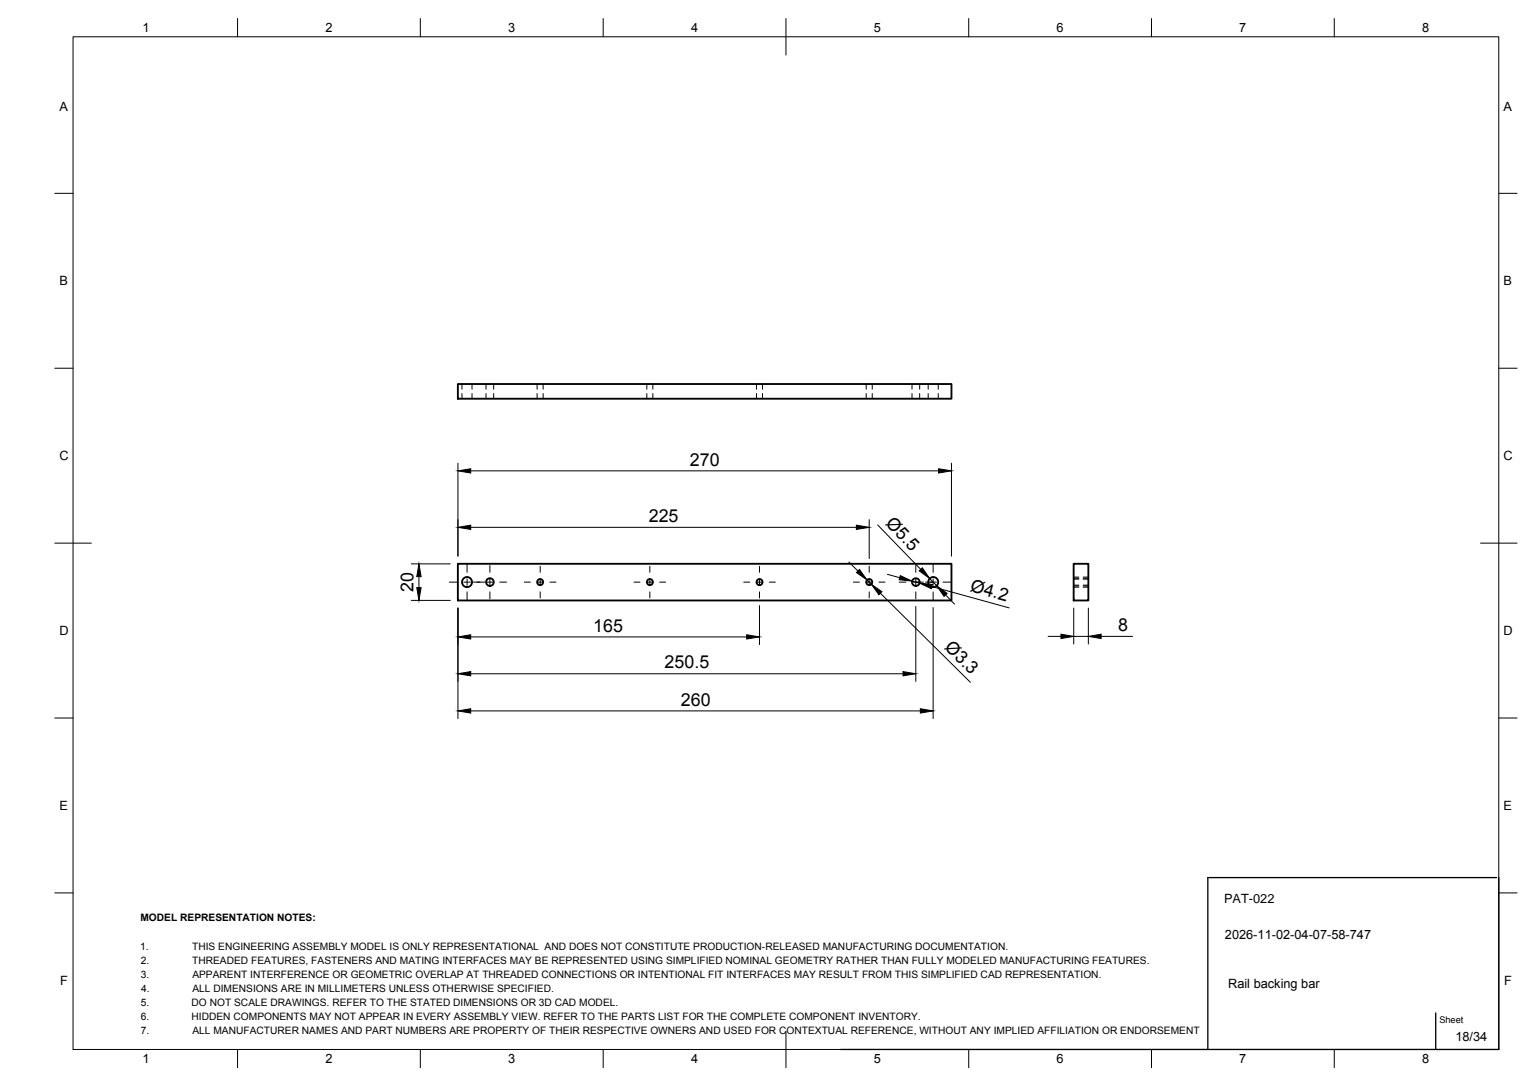
ISO-10303-21;
HEADER;
/* Generated by software containing ST-Developer
 * from STEP Tools, Inc. (www.steptools.com) 
 */

FILE_DESCRIPTION(
/* description */ ('Chute with adjustable gate'),
/* implementation_level */ '2;1');

FILE_NAME(
/* name */ 'Rail backing bar.step',
/* time_stamp */ '2026-10-27T10:52:28-07:00',
/* author */ (''),
/* organization */ (''),
/* preprocessor_version */ 'ST-DEVELOPER v20.2',
/* originating_system */ 'Autodesk Translation Framework v15.17.0.0',
/* authorisation */ '');

FILE_SCHEMA (('AUTOMOTIVE_DESIGN { 1 0 10303 214 3 1 1 }'));
ENDSEC;

DATA;
#10=MECHANICAL_DESIGN_GEOMETRIC_PRESENTATION_REPRESENTATION('',(#427),#13094);
#363=SHAPE_REPRESENTATION_RELATIONSHIP('SRR','None',#13264,#395);
#395=ADVANCED_BREP_SHAPE_REPRESENTATION('',(#459),#13073);
#427=STYLED_ITEM('',(#13481),#459);
#459=MANIFOLD_SOLID_BREP('Body1',#7610);
#520=FACE_BOUND('',#1507,.T.);
#521=FACE_BOUND('',#1508,.T.);
#522=FACE_BOUND('',#1509,.T.);
#523=FACE_BOUND('',#1510,.T.);
#524=FACE_BOUND('',#1511,.T.);
#525=FACE_BOUND('',#1512,.T.);
#526=FACE_BOUND('',#1513,.T.);
#527=FACE_BOUND('',#1514,.T.);
#528=FACE_BOUND('',#1517,.T.);
#529=FACE_BOUND('',#1518,.T.);
#530=FACE_BOUND('',#1519,.T.);
#531=FACE_BOUND('',#1520,.T.);
#532=FACE_BOUND('',#1521,.T.);
#533=FACE_BOUND('',#1522,.T.);
#534=FACE_BOUND('',#1523,.T.);
#535=FACE_BOUND('',#1524,.T.);
#688=PLANE('',#8196);
#689=PLANE('',#8197);
#690=PLANE('',#8198);
#691=PLANE('',#8199);
#692=PLANE('',#8200);
#693=PLANE('',#8201);
#1036=FACE_OUTER_BOUND('',#1497,.T.);
#1037=FACE_OUTER_BOUND('',#1498,.T.);
#1038=FACE_OUTER_BOUND('',#1499,.T.);
#1039=FACE_OUTER_BOUND('',#1500,.T.);
#1040=FACE_OUTER_BOUND('',#1501,.T.);
#1041=FACE_OUTER_BOUND('',#1502,.T.);
#1042=FACE_OUTER_BOUND('',#1503,.T.);
#1043=FACE_OUTER_BOUND('',#1504,.T.);
#1044=FACE_OUTER_BOUND('',#1505,.T.);
#1045=FACE_OUTER_BOUND('',#1506,.T.);
#1046=FACE_OUTER_BOUND('',#1515,.T.);
#1047=FACE_OUTER_BOUND('',#1516,.T.);
#1048=FACE_OUTER_BOUND('',#1525,.T.);
#1049=FACE_OUTER_BOUND('',#1526,.T.);
#1497=EDGE_LOOP('',(#5714,#5715,#5716,#5717));
#1498=EDGE_LOOP('',(#5718,#5719,#5720,#5721));
#1499=EDGE_LOOP('',(#5722,#5723,#5724,#5725));
#1500=EDGE_LOOP('',(#5726,#5727,#5728,#5729));
#1501=EDGE_LOOP('',(#5730,#5731,#5732,#5733));
#1502=EDGE_LOOP('',(#5734,#5735,#5736,#5737));
#1503=EDGE_LOOP('',(#5738,#5739,#5740,#5741));
#1504=EDGE_LOOP('',(#5742,#5743,#5744,#5745));
#1505=EDGE_LOOP('',(#5746,#5747,#5748,#5749));
#1506=EDGE_LOOP('',(#5750,#5751,#5752,#5753));
#1507=EDGE_LOOP('',(#5754));
#1508=EDGE_LOOP('',(#5755));
#1509=EDGE_LOOP('',(#5756));
#1510=EDGE_LOOP('',(#5757));
#1511=EDGE_LOOP('',(#5758));
#1512=EDGE_LOOP('',(#5759));
#1513=EDGE_LOOP('',(#5760));
#1514=EDGE_LOOP('',(#5761));
#1515=EDGE_LOOP('',(#5762,#5763,#5764,#5765));
#1516=EDGE_LOOP('',(#5766,#5767,#5768,#5769));
#1517=EDGE_LOOP('',(#5770));
#1518=EDGE_LOOP('',(#5771));
#1519=EDGE_LOOP('',(#5772));
#1520=EDGE_LOOP('',(#5773));
#1521=EDGE_LOOP('',(#5774));
#1522=EDGE_LOOP('',(#5775));
#1523=EDGE_LOOP('',(#5776));
#1524=EDGE_LOOP('',(#5777));
#1525=EDGE_LOOP('',(#5778,#5779,#5780,#5781));
#1526=EDGE_LOOP('',(#5782,#5783,#5784,#5785));
#2076=LINE('',#11481,#2853);
#2077=LINE('',#11487,#2854);
#2078=LINE('',#11493,#2855);
#2079=LINE('',#11499,#2856);
#2080=LINE('',#11505,#2857);
#2081=LINE('',#11511,#2858);
#2082=LINE('',#11517,#2859);
#2083=LINE('',#11523,#2860);
#2084=LINE('',#11528,#2861);
#2085=LINE('',#11530,#2862);
#2086=LINE('',#11532,#2863);
#2087=LINE('',#11533,#2864);
#2088=LINE('',#11536,#2865);
#2089=LINE('',#11538,#2866);
#2090=LINE('',#11539,#2867);
#2091=LINE('',#11542,#2868);
#2092=LINE('',#11544,#2869);
#2093=LINE('',#11545,#2870);
#2094=LINE('',#11547,#2871);
#2095=LINE('',#11548,#2872);
#2853=VECTOR('',#9290,0.210000000000001);
#2854=VECTOR('',#9297,0.21);
#2855=VECTOR('',#9304,0.164999999999999);
#2856=VECTOR('',#9311,0.164999999999999);
#2857=VECTOR('',#9318,0.164999999999999);
#2858=VECTOR('',#9325,0.164999999999999);
#2859=VECTOR('',#9332,0.275);
#2860=VECTOR('',#9339,0.274999999999999);
#2861=VECTOR('',#9344,1.);
#2862=VECTOR('',#9345,1.);
#2863=VECTOR('',#9346,1.);
#2864=VECTOR('',#9347,1.);
#2865=VECTOR('',#9350,1.);
#2866=VECTOR('',#9351,1.);
#2867=VECTOR('',#9352,1.);
#2868=VECTOR('',#9355,1.);
#2869=VECTOR('',#9356,1.);
#2870=VECTOR('',#9357,1.);
#2871=VECTOR('',#9360,1.);
#2872=VECTOR('',#9361,1.);
#3462=CIRCLE('',#8173,0.210000000000001);
#3463=CIRCLE('',#8174,0.210000000000001);
#3464=CIRCLE('',#8176,0.21);
#3465=CIRCLE('',#8177,0.21);
#3466=CIRCLE('',#8179,0.164999999999999);
#3467=CIRCLE('',#8180,0.164999999999999);
#3468=CIRCLE('',#8182,0.164999999999999);
#3469=CIRCLE('',#8183,0.164999999999999);
#3470=CIRCLE('',#8185,0.164999999999999);
#3471=CIRCLE('',#8186,0.164999999999999);
#3472=CIRCLE('',#8188,0.164999999999999);
#3473=CIRCLE('',#8189,0.164999999999999);
#3474=CIRCLE('',#8191,0.275);
#3475=CIRCLE('',#8192,0.275);
#3476=CIRCLE('',#8194,0.274999999999999);
#3477=CIRCLE('',#8195,0.274999999999999);
#3769=VERTEX_POINT('',#11478);
#3770=VERTEX_POINT('',#11480);
#3771=VERTEX_POINT('',#11484);
#3772=VERTEX_POINT('',#11486);
#3773=VERTEX_POINT('',#11490);
#3774=VERTEX_POINT('',#11492);
#3775=VERTEX_POINT('',#11496);
#3776=VERTEX_POINT('',#11498);
#3777=VERTEX_POINT('',#11502);
#3778=VERTEX_POINT('',#11504);
#3779=VERTEX_POINT('',#11508);
#3780=VERTEX_POINT('',#11510);
#3781=VERTEX_POINT('',#11514);
#3782=VERTEX_POINT('',#11516);
#3783=VERTEX_POINT('',#11520);
#3784=VERTEX_POINT('',#11522);
#3785=VERTEX_POINT('',#11526);
#3786=VERTEX_POINT('',#11527);
#3787=VERTEX_POINT('',#11529);
#3788=VERTEX_POINT('',#11531);
#3789=VERTEX_POINT('',#11535);
#3790=VERTEX_POINT('',#11537);
#3791=VERTEX_POINT('',#11541);
#3792=VERTEX_POINT('',#11543);
#4490=EDGE_CURVE('',#3769,#3769,#3462,.T.);
#4491=EDGE_CURVE('',#3769,#3770,#2076,.T.);
#4492=EDGE_CURVE('',#3770,#3770,#3463,.T.);
#4493=EDGE_CURVE('',#3771,#3771,#3464,.T.);
#4494=EDGE_CURVE('',#3771,#3772,#2077,.T.);
#4495=EDGE_CURVE('',#3772,#3772,#3465,.T.);
#4496=EDGE_CURVE('',#3773,#3773,#3466,.T.);
#4497=EDGE_CURVE('',#3773,#3774,#2078,.T.);
#4498=EDGE_CURVE('',#3774,#3774,#3467,.T.);
#4499=EDGE_CURVE('',#3775,#3775,#3468,.T.);
#4500=EDGE_CURVE('',#3775,#3776,#2079,.T.);
#4501=EDGE_CURVE('',#3776,#3776,#3469,.T.);
#4502=EDGE_CURVE('',#3777,#3777,#3470,.T.);
#4503=EDGE_CURVE('',#3777,#3778,#2080,.T.);
#4504=EDGE_CURVE('',#3778,#3778,#3471,.T.);
#4505=EDGE_CURVE('',#3779,#3779,#3472,.T.);
#4506=EDGE_CURVE('',#3779,#3780,#2081,.T.);
#4507=EDGE_CURVE('',#3780,#3780,#3473,.T.);
#4508=EDGE_CURVE('',#3781,#3781,#3474,.T.);
#4509=EDGE_CURVE('',#3781,#3782,#2082,.T.);
#4510=EDGE_CURVE('',#3782,#3782,#3475,.T.);
#4511=EDGE_CURVE('',#3783,#3783,#3476,.T.);
#4512=EDGE_CURVE('',#3783,#3784,#2083,.T.);
#4513=EDGE_CURVE('',#3784,#3784,#3477,.T.);
#4514=EDGE_CURVE('',#3785,#3786,#2084,.T.);
#4515=EDGE_CURVE('',#3786,#3787,#2085,.T.);
#4516=EDGE_CURVE('',#3788,#3787,#2086,.T.);
#4517=EDGE_CURVE('',#3785,#3788,#2087,.T.);
#4518=EDGE_CURVE('',#3789,#3785,#2088,.T.);
#4519=EDGE_CURVE('',#3790,#3788,#2089,.T.);
#4520=EDGE_CURVE('',#3789,#3790,#2090,.T.);
#4521=EDGE_CURVE('',#3791,#3789,#2091,.T.);
#4522=EDGE_CURVE('',#3792,#3790,#2092,.T.);
#4523=EDGE_CURVE('',#3791,#3792,#2093,.T.);
#4524=EDGE_CURVE('',#3786,#3791,#2094,.T.);
#4525=EDGE_CURVE('',#3787,#3792,#2095,.T.);
#5714=ORIENTED_EDGE('',*,*,#4490,.F.);
#5715=ORIENTED_EDGE('',*,*,#4491,.T.);
#5716=ORIENTED_EDGE('',*,*,#4492,.F.);
#5717=ORIENTED_EDGE('',*,*,#4491,.F.);
#5718=ORIENTED_EDGE('',*,*,#4493,.F.);
#5719=ORIENTED_EDGE('',*,*,#4494,.T.);
#5720=ORIENTED_EDGE('',*,*,#4495,.F.);
#5721=ORIENTED_EDGE('',*,*,#4494,.F.);
#5722=ORIENTED_EDGE('',*,*,#4496,.F.);
#5723=ORIENTED_EDGE('',*,*,#4497,.T.);
#5724=ORIENTED_EDGE('',*,*,#4498,.F.);
#5725=ORIENTED_EDGE('',*,*,#4497,.F.);
#5726=ORIENTED_EDGE('',*,*,#4499,.F.);
#5727=ORIENTED_EDGE('',*,*,#4500,.T.);
#5728=ORIENTED_EDGE('',*,*,#4501,.F.);
#5729=ORIENTED_EDGE('',*,*,#4500,.F.);
#5730=ORIENTED_EDGE('',*,*,#4502,.F.);
#5731=ORIENTED_EDGE('',*,*,#4503,.T.);
#5732=ORIENTED_EDGE('',*,*,#4504,.F.);
#5733=ORIENTED_EDGE('',*,*,#4503,.F.);
#5734=ORIENTED_EDGE('',*,*,#4505,.F.);
#5735=ORIENTED_EDGE('',*,*,#4506,.T.);
#5736=ORIENTED_EDGE('',*,*,#4507,.F.);
#5737=ORIENTED_EDGE('',*,*,#4506,.F.);
#5738=ORIENTED_EDGE('',*,*,#4508,.F.);
#5739=ORIENTED_EDGE('',*,*,#4509,.T.);
#5740=ORIENTED_EDGE('',*,*,#4510,.F.);
#5741=ORIENTED_EDGE('',*,*,#4509,.F.);
#5742=ORIENTED_EDGE('',*,*,#4511,.F.);
#5743=ORIENTED_EDGE('',*,*,#4512,.T.);
#5744=ORIENTED_EDGE('',*,*,#4513,.F.);
#5745=ORIENTED_EDGE('',*,*,#4512,.F.);
#5746=ORIENTED_EDGE('',*,*,#4514,.T.);
#5747=ORIENTED_EDGE('',*,*,#4515,.T.);
#5748=ORIENTED_EDGE('',*,*,#4516,.F.);
#5749=ORIENTED_EDGE('',*,*,#4517,.F.);
#5750=ORIENTED_EDGE('',*,*,#4518,.T.);
#5751=ORIENTED_EDGE('',*,*,#4517,.T.);
#5752=ORIENTED_EDGE('',*,*,#4519,.F.);
#5753=ORIENTED_EDGE('',*,*,#4520,.F.);
#5754=ORIENTED_EDGE('',*,*,#4498,.T.);
#5755=ORIENTED_EDGE('',*,*,#4501,.T.);
#5756=ORIENTED_EDGE('',*,*,#4504,.T.);
#5757=ORIENTED_EDGE('',*,*,#4507,.T.);
#5758=ORIENTED_EDGE('',*,*,#4510,.T.);
#5759=ORIENTED_EDGE('',*,*,#4513,.T.);
#5760=ORIENTED_EDGE('',*,*,#4495,.T.);
#5761=ORIENTED_EDGE('',*,*,#4492,.T.);
#5762=ORIENTED_EDGE('',*,*,#4521,.T.);
#5763=ORIENTED_EDGE('',*,*,#4520,.T.);
#5764=ORIENTED_EDGE('',*,*,#4522,.F.);
#5765=ORIENTED_EDGE('',*,*,#4523,.F.);
#5766=ORIENTED_EDGE('',*,*,#4524,.T.);
#5767=ORIENTED_EDGE('',*,*,#4523,.T.);
#5768=ORIENTED_EDGE('',*,*,#4525,.F.);
#5769=ORIENTED_EDGE('',*,*,#4515,.F.);
#5770=ORIENTED_EDGE('',*,*,#4496,.T.);
#5771=ORIENTED_EDGE('',*,*,#4499,.T.);
#5772=ORIENTED_EDGE('',*,*,#4502,.T.);
#5773=ORIENTED_EDGE('',*,*,#4505,.T.);
#5774=ORIENTED_EDGE('',*,*,#4508,.T.);
#5775=ORIENTED_EDGE('',*,*,#4511,.T.);
#5776=ORIENTED_EDGE('',*,*,#4493,.T.);
#5777=ORIENTED_EDGE('',*,*,#4490,.T.);
#5778=ORIENTED_EDGE('',*,*,#4525,.T.);
#5779=ORIENTED_EDGE('',*,*,#4522,.T.);
#5780=ORIENTED_EDGE('',*,*,#4519,.T.);
#5781=ORIENTED_EDGE('',*,*,#4516,.T.);
#5782=ORIENTED_EDGE('',*,*,#4524,.F.);
#5783=ORIENTED_EDGE('',*,*,#4514,.F.);
#5784=ORIENTED_EDGE('',*,*,#4518,.F.);
#5785=ORIENTED_EDGE('',*,*,#4521,.F.);
#7130=CYLINDRICAL_SURFACE('',#8172,0.210000000000001);
#7131=CYLINDRICAL_SURFACE('',#8175,0.21);
#7132=CYLINDRICAL_SURFACE('',#8178,0.164999999999999);
#7133=CYLINDRICAL_SURFACE('',#8181,0.164999999999999);
#7134=CYLINDRICAL_SURFACE('',#8184,0.164999999999999);
#7135=CYLINDRICAL_SURFACE('',#8187,0.164999999999999);
#7136=CYLINDRICAL_SURFACE('',#8190,0.275);
#7137=CYLINDRICAL_SURFACE('',#8193,0.274999999999999);
#7304=ADVANCED_FACE('',(#1036),#7130,.F.);
#7305=ADVANCED_FACE('',(#1037),#7131,.F.);
#7306=ADVANCED_FACE('',(#1038),#7132,.F.);
#7307=ADVANCED_FACE('',(#1039),#7133,.F.);
#7308=ADVANCED_FACE('',(#1040),#7134,.F.);
#7309=ADVANCED_FACE('',(#1041),#7135,.F.);
#7310=ADVANCED_FACE('',(#1042),#7136,.F.);
#7311=ADVANCED_FACE('',(#1043),#7137,.F.);
#7312=ADVANCED_FACE('',(#1044),#688,.T.);
#7313=ADVANCED_FACE('',(#1045,#520,#521,#522,#523,#524,#525,#526,#527),
#689,.T.);
#7314=ADVANCED_FACE('',(#1046),#690,.T.);
#7315=ADVANCED_FACE('',(#1047,#528,#529,#530,#531,#532,#533,#534,#535),
#691,.T.);
#7316=ADVANCED_FACE('',(#1048),#692,.T.);
#7317=ADVANCED_FACE('',(#1049),#693,.F.);
#7610=CLOSED_SHELL('',(#7304,#7305,#7306,#7307,#7308,#7309,#7310,#7311,
#7312,#7313,#7314,#7315,#7316,#7317));
#8171=AXIS2_PLACEMENT_3D('',#11476,#9284,#9285);
#8172=AXIS2_PLACEMENT_3D('',#11477,#9286,#9287);
#8173=AXIS2_PLACEMENT_3D('',#11479,#9288,#9289);
#8174=AXIS2_PLACEMENT_3D('',#11482,#9291,#9292);
#8175=AXIS2_PLACEMENT_3D('',#11483,#9293,#9294);
#8176=AXIS2_PLACEMENT_3D('',#11485,#9295,#9296);
#8177=AXIS2_PLACEMENT_3D('',#11488,#9298,#9299);
#8178=AXIS2_PLACEMENT_3D('',#11489,#9300,#9301);
#8179=AXIS2_PLACEMENT_3D('',#11491,#9302,#9303);
#8180=AXIS2_PLACEMENT_3D('',#11494,#9305,#9306);
#8181=AXIS2_PLACEMENT_3D('',#11495,#9307,#9308);
#8182=AXIS2_PLACEMENT_3D('',#11497,#9309,#9310);
#8183=AXIS2_PLACEMENT_3D('',#11500,#9312,#9313);
#8184=AXIS2_PLACEMENT_3D('',#11501,#9314,#9315);
#8185=AXIS2_PLACEMENT_3D('',#11503,#9316,#9317);
#8186=AXIS2_PLACEMENT_3D('',#11506,#9319,#9320);
#8187=AXIS2_PLACEMENT_3D('',#11507,#9321,#9322);
#8188=AXIS2_PLACEMENT_3D('',#11509,#9323,#9324);
#8189=AXIS2_PLACEMENT_3D('',#11512,#9326,#9327);
#8190=AXIS2_PLACEMENT_3D('',#11513,#9328,#9329);
#8191=AXIS2_PLACEMENT_3D('',#11515,#9330,#9331);
#8192=AXIS2_PLACEMENT_3D('',#11518,#9333,#9334);
#8193=AXIS2_PLACEMENT_3D('',#11519,#9335,#9336);
#8194=AXIS2_PLACEMENT_3D('',#11521,#9337,#9338);
#8195=AXIS2_PLACEMENT_3D('',#11524,#9340,#9341);
#8196=AXIS2_PLACEMENT_3D('',#11525,#9342,#9343);
#8197=AXIS2_PLACEMENT_3D('',#11534,#9348,#9349);
#8198=AXIS2_PLACEMENT_3D('',#11540,#9353,#9354);
#8199=AXIS2_PLACEMENT_3D('',#11546,#9358,#9359);
#8200=AXIS2_PLACEMENT_3D('',#11549,#9362,#9363);
#8201=AXIS2_PLACEMENT_3D('',#11550,#9364,#9365);
#9284=DIRECTION('axis',(0.,0.,1.));
#9285=DIRECTION('refdir',(1.,0.,0.));
#9286=DIRECTION('center_axis',(1.,0.,0.));
#9287=DIRECTION('ref_axis',(0.,0.,-1.));
#9288=DIRECTION('center_axis',(1.,0.,0.));
#9289=DIRECTION('ref_axis',(0.,0.,-1.));
#9290=DIRECTION('',(1.,0.,0.));
#9291=DIRECTION('center_axis',(-1.,0.,0.));
#9292=DIRECTION('ref_axis',(0.,0.,-1.));
#9293=DIRECTION('center_axis',(1.,0.,0.));
#9294=DIRECTION('ref_axis',(0.,0.,-1.));
#9295=DIRECTION('center_axis',(1.,0.,0.));
#9296=DIRECTION('ref_axis',(0.,0.,-1.));
#9297=DIRECTION('',(1.,0.,0.));
#9298=DIRECTION('center_axis',(-1.,0.,0.));
#9299=DIRECTION('ref_axis',(0.,0.,-1.));
#9300=DIRECTION('center_axis',(1.,0.,0.));
#9301=DIRECTION('ref_axis',(0.,0.,-1.));
#9302=DIRECTION('center_axis',(1.,0.,0.));
#9303=DIRECTION('ref_axis',(0.,0.,-1.));
#9304=DIRECTION('',(1.,0.,0.));
#9305=DIRECTION('center_axis',(-1.,0.,0.));
#9306=DIRECTION('ref_axis',(0.,0.,-1.));
#9307=DIRECTION('center_axis',(1.,0.,0.));
#9308=DIRECTION('ref_axis',(0.,0.,-1.));
#9309=DIRECTION('center_axis',(1.,0.,0.));
#9310=DIRECTION('ref_axis',(0.,0.,-1.));
#9311=DIRECTION('',(1.,0.,0.));
#9312=DIRECTION('center_axis',(-1.,0.,0.));
#9313=DIRECTION('ref_axis',(0.,0.,-1.));
#9314=DIRECTION('center_axis',(1.,0.,0.));
#9315=DIRECTION('ref_axis',(0.,0.,-1.));
#9316=DIRECTION('center_axis',(1.,0.,0.));
#9317=DIRECTION('ref_axis',(0.,0.,-1.));
#9318=DIRECTION('',(1.,0.,0.));
#9319=DIRECTION('center_axis',(-1.,0.,0.));
#9320=DIRECTION('ref_axis',(0.,0.,-1.));
#9321=DIRECTION('center_axis',(1.,0.,0.));
#9322=DIRECTION('ref_axis',(0.,0.,-1.));
#9323=DIRECTION('center_axis',(1.,0.,0.));
#9324=DIRECTION('ref_axis',(0.,0.,-1.));
#9325=DIRECTION('',(1.,0.,0.));
#9326=DIRECTION('center_axis',(-1.,0.,0.));
#9327=DIRECTION('ref_axis',(0.,0.,-1.));
#9328=DIRECTION('center_axis',(1.,0.,0.));
#9329=DIRECTION('ref_axis',(0.,0.,-1.));
#9330=DIRECTION('center_axis',(1.,0.,0.));
#9331=DIRECTION('ref_axis',(0.,0.,-1.));
#9332=DIRECTION('',(1.,0.,0.));
#9333=DIRECTION('center_axis',(-1.,0.,0.));
#9334=DIRECTION('ref_axis',(0.,0.,-1.));
#9335=DIRECTION('center_axis',(1.,0.,0.));
#9336=DIRECTION('ref_axis',(0.,0.,-1.));
#9337=DIRECTION('center_axis',(1.,0.,0.));
#9338=DIRECTION('ref_axis',(0.,0.,-1.));
#9339=DIRECTION('',(1.,0.,0.));
#9340=DIRECTION('center_axis',(-1.,0.,0.));
#9341=DIRECTION('ref_axis',(0.,0.,-1.));
#9342=DIRECTION('center_axis',(0.,1.,0.));
#9343=DIRECTION('ref_axis',(-1.,0.,0.));
#9344=DIRECTION('',(-1.,0.,0.));
#9345=DIRECTION('',(0.,0.,1.));
#9346=DIRECTION('',(-1.,0.,0.));
#9347=DIRECTION('',(0.,0.,1.));
#9348=DIRECTION('center_axis',(1.,0.,0.));
#9349=DIRECTION('ref_axis',(0.,1.,0.));
#9350=DIRECTION('',(0.,1.,0.));
#9351=DIRECTION('',(0.,1.,0.));
#9352=DIRECTION('',(0.,0.,1.));
#9353=DIRECTION('center_axis',(0.,-1.,0.));
#9354=DIRECTION('ref_axis',(1.,0.,0.));
#9355=DIRECTION('',(1.,0.,0.));
#9356=DIRECTION('',(1.,0.,0.));
#9357=DIRECTION('',(0.,0.,1.));
#9358=DIRECTION('center_axis',(-1.,0.,0.));
#9359=DIRECTION('ref_axis',(0.,-1.,0.));
#9360=DIRECTION('',(0.,-1.,0.));
#9361=DIRECTION('',(0.,-1.,0.));
#9362=DIRECTION('center_axis',(0.,0.,1.));
#9363=DIRECTION('ref_axis',(1.,0.,0.));
#9364=DIRECTION('center_axis',(0.,0.,1.));
#9365=DIRECTION('ref_axis',(1.,0.,0.));
#11476=CARTESIAN_POINT('',(0.,0.,0.));
#11477=CARTESIAN_POINT('Origin',(1.1,11.,30.25));
#11478=CARTESIAN_POINT('',(1.2,11.,30.46));
#11479=CARTESIAN_POINT('Origin',(1.2,11.,30.25));
#11480=CARTESIAN_POINT('',(2.,11.,30.46));
#11481=CARTESIAN_POINT('',(1.1,11.,30.46));
#11482=CARTESIAN_POINT('Origin',(2.,11.,30.25));
#11483=CARTESIAN_POINT('Origin',(1.1,11.,6.95));
#11484=CARTESIAN_POINT('',(1.2,11.,7.16));
#11485=CARTESIAN_POINT('Origin',(1.2,11.,6.95));
#11486=CARTESIAN_POINT('',(2.,11.,7.16));
#11487=CARTESIAN_POINT('',(1.1,11.,7.16));
#11488=CARTESIAN_POINT('Origin',(2.,11.,6.95));
#11489=CARTESIAN_POINT('Origin',(1.1,11.,21.5));
#11490=CARTESIAN_POINT('',(1.2,11.,21.665));
#11491=CARTESIAN_POINT('Origin',(1.2,11.,21.5));
#11492=CARTESIAN_POINT('',(2.,11.,21.665));
#11493=CARTESIAN_POINT('',(1.1,11.,21.665));
#11494=CARTESIAN_POINT('Origin',(2.,11.,21.5));
#11495=CARTESIAN_POINT('Origin',(1.1,11.,15.5));
#11496=CARTESIAN_POINT('',(1.2,11.,15.665));
#11497=CARTESIAN_POINT('Origin',(1.2,11.,15.5));
#11498=CARTESIAN_POINT('',(2.,11.,15.665));
#11499=CARTESIAN_POINT('',(1.1,11.,15.665));
#11500=CARTESIAN_POINT('Origin',(2.,11.,15.5));
#11501=CARTESIAN_POINT('Origin',(1.1,11.,9.5));
#11502=CARTESIAN_POINT('',(1.2,11.,9.665));
#11503=CARTESIAN_POINT('Origin',(1.2,11.,9.5));
#11504=CARTESIAN_POINT('',(2.,11.,9.665));
#11505=CARTESIAN_POINT('',(1.1,11.,9.665));
#11506=CARTESIAN_POINT('Origin',(2.,11.,9.5));
#11507=CARTESIAN_POINT('Origin',(1.1,11.,27.5));
#11508=CARTESIAN_POINT('',(1.2,11.,27.665));
#11509=CARTESIAN_POINT('Origin',(1.2,11.,27.5));
#11510=CARTESIAN_POINT('',(2.,11.,27.665));
#11511=CARTESIAN_POINT('',(1.1,11.,27.665));
#11512=CARTESIAN_POINT('Origin',(2.,11.,27.5));
#11513=CARTESIAN_POINT('Origin',(1.1,11.,6.));
#11514=CARTESIAN_POINT('',(1.2,11.,6.275));
#11515=CARTESIAN_POINT('Origin',(1.2,11.,6.));
#11516=CARTESIAN_POINT('',(2.,11.,6.275));
#11517=CARTESIAN_POINT('',(1.1,11.,6.275));
#11518=CARTESIAN_POINT('Origin',(2.,11.,6.));
#11519=CARTESIAN_POINT('Origin',(1.1,11.,31.5));
#11520=CARTESIAN_POINT('',(1.2,11.,31.775));
#11521=CARTESIAN_POINT('Origin',(1.2,11.,31.5));
#11522=CARTESIAN_POINT('',(2.,11.,31.775));
#11523=CARTESIAN_POINT('',(1.1,11.,31.775));
#11524=CARTESIAN_POINT('Origin',(2.,11.,31.5));
#11525=CARTESIAN_POINT('Origin',(2.,12.,5.));
#11526=CARTESIAN_POINT('',(2.,12.,5.));
#11527=CARTESIAN_POINT('',(1.2,12.,5.));
#11528=CARTESIAN_POINT('',(2.,12.,5.));
#11529=CARTESIAN_POINT('',(1.2,12.,32.));
#11530=CARTESIAN_POINT('',(1.2,12.,5.));
#11531=CARTESIAN_POINT('',(2.,12.,32.));
#11532=CARTESIAN_POINT('',(2.,12.,32.));
#11533=CARTESIAN_POINT('',(2.,12.,5.));
#11534=CARTESIAN_POINT('Origin',(2.,10.,5.));
#11535=CARTESIAN_POINT('',(2.,10.,5.));
#11536=CARTESIAN_POINT('',(2.,10.,5.));
#11537=CARTESIAN_POINT('',(2.,10.,32.));
#11538=CARTESIAN_POINT('',(2.,10.,32.));
#11539=CARTESIAN_POINT('',(2.,10.,5.));
#11540=CARTESIAN_POINT('Origin',(1.2,10.,5.));
#11541=CARTESIAN_POINT('',(1.2,10.,5.));
#11542=CARTESIAN_POINT('',(1.2,10.,5.));
#11543=CARTESIAN_POINT('',(1.2,10.,32.));
#11544=CARTESIAN_POINT('',(1.2,10.,32.));
#11545=CARTESIAN_POINT('',(1.2,10.,5.));
#11546=CARTESIAN_POINT('Origin',(1.2,12.,5.));
#11547=CARTESIAN_POINT('',(1.2,12.,5.));
#11548=CARTESIAN_POINT('',(1.2,12.,32.));
#11549=CARTESIAN_POINT('Origin',(1.6,11.,32.));
#11550=CARTESIAN_POINT('Origin',(1.6,11.,5.));
#13036=UNCERTAINTY_MEASURE_WITH_UNIT(LENGTH_MEASURE(0.001),#13095,
'DISTANCE_ACCURACY_VALUE',
'Maximum model space distance between geometric entities at asserted c
onnectivities');
#13057=UNCERTAINTY_MEASURE_WITH_UNIT(LENGTH_MEASURE(0.001),#13095,
'DISTANCE_ACCURACY_VALUE',
'Maximum model space distance between geometric entities at asserted c
onnectivities');
#13073=(
GEOMETRIC_REPRESENTATION_CONTEXT(3)
GLOBAL_UNCERTAINTY_ASSIGNED_CONTEXT((#13036))
GLOBAL_UNIT_ASSIGNED_CONTEXT((#13095,#13097,#13098))
REPRESENTATION_CONTEXT('','3D')
);
#13094=(
GEOMETRIC_REPRESENTATION_CONTEXT(3)
GLOBAL_UNCERTAINTY_ASSIGNED_CONTEXT((#13057))
GLOBAL_UNIT_ASSIGNED_CONTEXT((#13095,#13097,#13098))
REPRESENTATION_CONTEXT('','3D')
);
#13095=(
LENGTH_UNIT()
NAMED_UNIT(*)
SI_UNIT(.CENTI.,.METRE.)
);
#13097=(
NAMED_UNIT(*)
PLANE_ANGLE_UNIT()
SI_UNIT($,.RADIAN.)
);
#13098=(
NAMED_UNIT(*)
SI_UNIT($,.STERADIAN.)
SOLID_ANGLE_UNIT()
);
#13114=SHAPE_DEFINITION_REPRESENTATION(#13150,#13264);
#13150=PRODUCT_DEFINITION_SHAPE('',$,#13301);
#13264=SHAPE_REPRESENTATION('',(#8171),#13073);
#13285=PRODUCT_DEFINITION_CONTEXT('part definition',#13395,'design');
#13301=PRODUCT_DEFINITION('Rail backing bar','Rail backing bar',#13337,
#13285);
#13337=PRODUCT_DEFINITION_FORMATION('',$,#13412);
#13395=APPLICATION_CONTEXT(
'Core Data for Automotive Mechanical Design Process');
#13396=PRODUCT_CONTEXT('part definition',#13395,'mechanical');
#13412=PRODUCT('Rail backing bar','Rail backing bar','Rail backing bar',
(#13396));
#13475=COLOUR_RGB('Light Blue',0.38,0.62,0.78);
#13476=FILL_AREA_STYLE_COLOUR('',#13475);
#13477=FILL_AREA_STYLE('',(#13476));
#13478=SURFACE_STYLE_FILL_AREA(#13477);
#13479=SURFACE_SIDE_STYLE('',(#13478));
#13480=SURFACE_STYLE_USAGE(.BOTH.,#13479);
#13481=PRESENTATION_STYLE_ASSIGNMENT((#13480));
ENDSEC;
END-ISO-10303-21;
